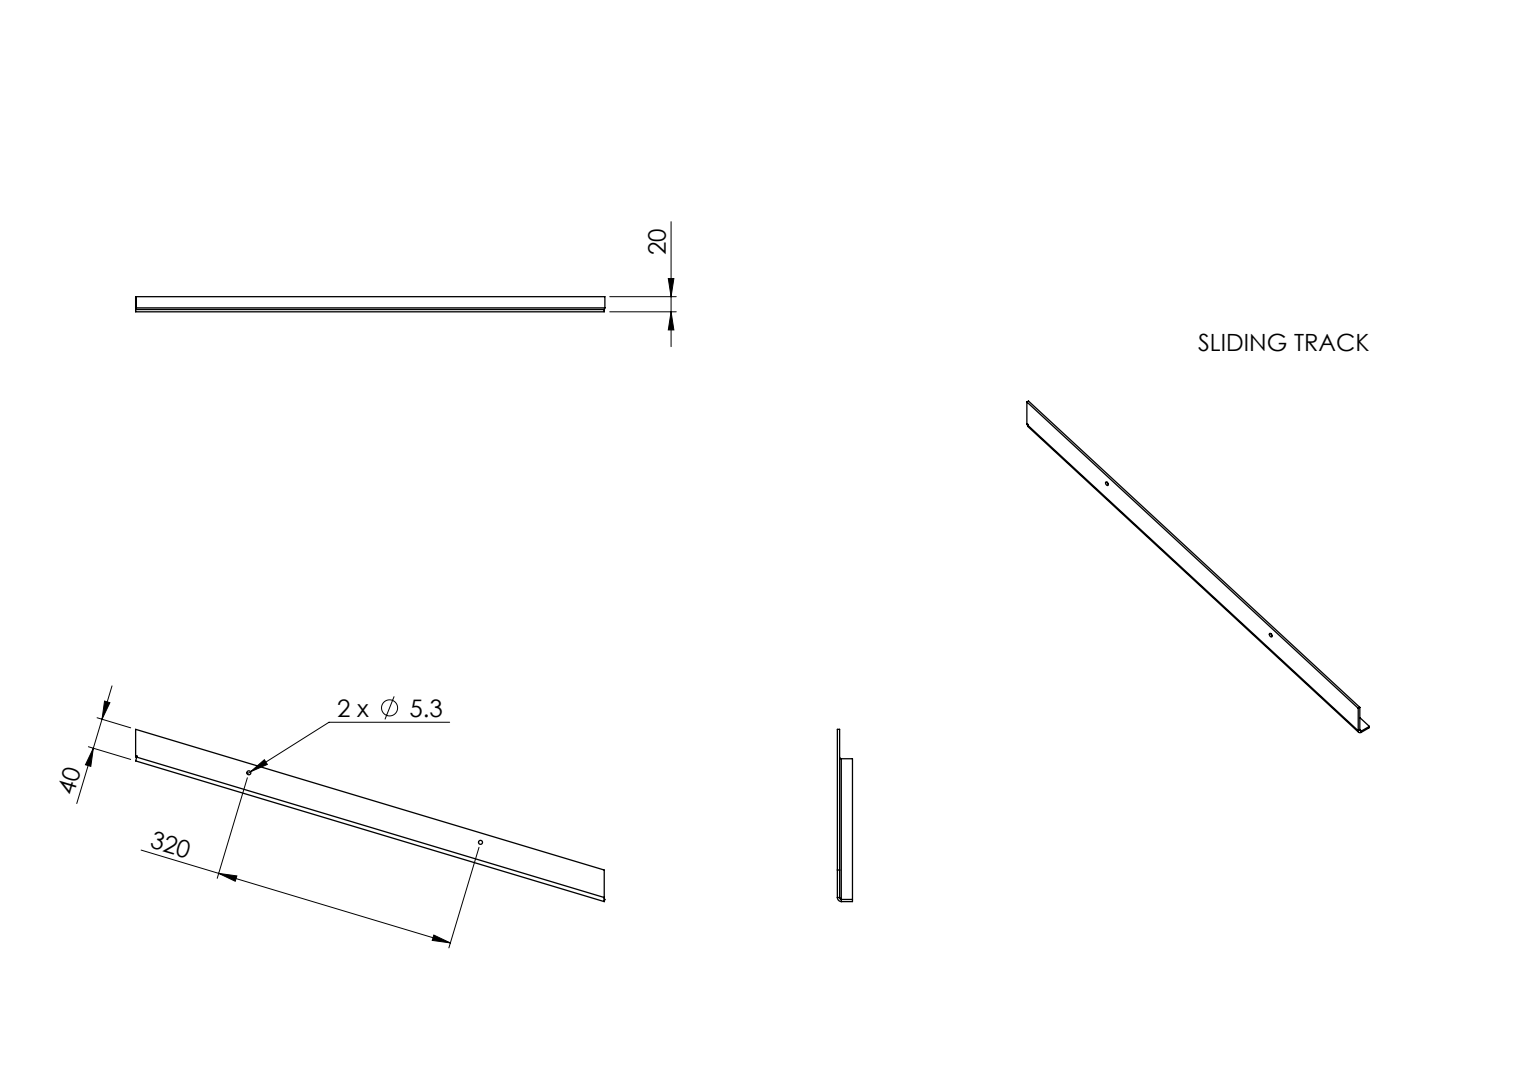
ISO-10303-21;
HEADER;
FILE_DESCRIPTION (('STEP AP214'),
    '1' );
FILE_NAME ('sliding track.step',
    '2026-10-27T17:01:19',
    ( '' ),
    ( '' ),
    'SwSTEP 2.0',
    'SolidWorks 2026',
    '' );
FILE_SCHEMA (( 'AUTOMOTIVE_DESIGN' ));
ENDSEC;

DATA;
#58=EDGE_CURVE ( 'NONE', #5396, #13410, #5058, .T. ) ;
#64=DIRECTION ( 'NONE',  ( 0.000000000000000000, 0.000000000000000000, 1.000000000000000000 ) ) ;
#77=EDGE_CURVE ( 'NONE', #2441, #3014, #1734, .T. ) ;
#96=SHAPE_REPRESENTATION_RELATIONSHIP ( 'NONE' , 'NONE' ,  #14430, #6538 ) ;
#102=ADVANCED_FACE ( 'NONE', ( #9327 ), #3935, .F. ) ;
#150=CARTESIAN_POINT ( 'NONE',  ( 142.4540310085880606, 355.9707293956415697, 187.0000000000000000 ) ) ;
#157=EDGE_CURVE ( 'NONE', #12209, #11318, #10435, .T. ) ;
#268=CARTESIAN_POINT ( 'NONE',  ( 610.0000000000001137, 185.6790804732684137, 184.8000000000000682 ) ) ;
#333=CARTESIAN_POINT ( 'NONE',  ( 609.8668404561643683, 185.6877074168924935, 185.4847245573741930 ) ) ;
#374=ORIENTED_EDGE ( 'NONE', *, *, #847, .F. ) ;
#378=DIRECTION ( 'NONE',  ( -1.000000000000000000, 0.000000000000000000, 0.000000000000000000 ) ) ;
#410=CARTESIAN_POINT ( 'NONE',  ( 609.6905198467529772, 186.4571330906553044, 187.4188186979287423 ) ) ;
#418=( GEOMETRIC_REPRESENTATION_CONTEXT ( 3 ) GLOBAL_UNCERTAINTY_ASSIGNED_CONTEXT ( ( #11082 ) ) GLOBAL_UNIT_ASSIGNED_CONTEXT ( ( #12770, #11436, #9372 ) ) REPRESENTATION_CONTEXT ( 'NONE', 'WORKASPACE' ) );
#467=DIRECTION ( 'NONE',  ( -0.9578262852211513190, 0.2873478855663453846, -8.575812866481462478E-17 ) ) ;
#511=DIRECTION ( 'NONE',  ( -1.000000000000000000, 0.000000000000000000, 0.000000000000000000 ) ) ;
#526=LINE ( 'NONE', #5051, #11486 ) ;
#558=CARTESIAN_POINT ( 'NONE',  ( 610.3687250539534261, 189.1718658564638247, 186.1427899493634470 ) ) ;
#572=ADVANCED_FACE ( 'NONE', ( #12850 ), #2893, .F. ) ;
#593=ORIENTED_EDGE ( 'NONE', *, *, #77, .F. ) ;
#627=CARTESIAN_POINT ( 'NONE',  ( -112.9080459801079144, 33.87241379403258890, 190.0000000000000000 ) ) ;
#629=CARTESIAN_POINT ( 'NONE',  ( 609.6990281814310038, 187.8427340524074225, 188.9822575857425022 ) ) ;
#644=VECTOR ( 'NONE', #4252, 1000.000000000000227 ) ;
#665=DIRECTION ( 'NONE',  ( -0.9578262852211518741, 0.2873478855663437748, 0.000000000000000000 ) ) ;
#688=AXIS2_PLACEMENT_3D ( 'NONE', #6223, #665, #7180 ) ;
#701=CARTESIAN_POINT ( 'NONE',  ( 610.0832774997078332, 190.4835367118463125, 186.9433982284626552 ) ) ;
#704=EDGE_CURVE ( 'NONE', #7308, #3640, #8632, .T. ) ;
#727=FACE_OUTER_BOUND ( 'NONE', #13601, .T. ) ;
#729=VECTOR ( 'NONE', #9292, 1000.000000000000000 ) ;
#743=CARTESIAN_POINT ( 'NONE',  ( 139.8040310085880833, 355.9707293956415697, 190.0000000000000000 ) ) ;
#847=EDGE_CURVE ( 'NONE', #13246, #3959, #4647, .T. ) ;
#913=CARTESIAN_POINT ( 'NONE',  ( 609.6836880993740806, 187.1145182921505921, 188.2379512264755874 ) ) ;
#933=AXIS2_PLACEMENT_3D ( 'NONE', #743, #5266, #12107 ) ;
#943=CARTESIAN_POINT ( 'NONE',  ( 610.0000000000000000, 227.4403065089105951, 187.0000000000000000 ) ) ;
#966=EDGE_CURVE ( 'NONE', #9351, #2398, #12904, .T. ) ;
#967=DIRECTION ( 'NONE',  ( -0.2873478855663452736, -0.9578262852211514300, 0.000000000000000000 ) ) ;
#979=ORIENTED_EDGE ( 'NONE', *, *, #13235, .T. ) ;
#981=CARTESIAN_POINT ( 'NONE',  ( 610.0000000000002274, 191.1080398579018720, 187.0000000000000284 ) ) ;
#983=VECTOR ( 'NONE', #4579, 1000.000000000000227 ) ;
#989=DIRECTION ( 'NONE',  ( 0.9578262852211513190, -0.2873478855663453846, -0.000000000000000000 ) ) ;
#993=CARTESIAN_POINT ( 'NONE',  ( 609.6939753585367043, 187.4861613156657540, 188.5968284039610978 ) ) ;
#1006=CARTESIAN_POINT ( 'NONE',  ( 610.1840840298345938, 189.9120001624725376, 186.6958543268122526 ) ) ;
#1011=EDGE_CURVE ( 'NONE', #2694, #5805, #12133, .T. ) ;
#1039=DIRECTION ( 'NONE',  ( 0.000000000000000000, -1.000000000000000000, 0.000000000000000000 ) ) ;
#1067=ORIENTED_EDGE ( 'NONE', *, *, #2953, .F. ) ;
#1077=( LENGTH_UNIT ( ) NAMED_UNIT ( * ) SI_UNIT ( .MILLI., .METRE. ) );
#1087=DIRECTION ( 'NONE',  ( -0.000000000000000000, 0.000000000000000000, 1.000000000000000000 ) ) ;
#1121=ORIENTED_EDGE ( 'NONE', *, *, #2407, .T. ) ;
#1142=AXIS2_PLACEMENT_3D ( 'NONE', #1745, #6320, #10822 ) ;
#1168=ORIENTED_EDGE ( 'NONE', *, *, #11531, .F. ) ;
#1171=PRODUCT_CONTEXT ( 'NONE', #13377, 'mechanical' ) ;
#1187=VECTOR ( 'NONE', #4576, 1000.000000000000000 ) ;
#1220=VECTOR ( 'NONE', #13865, 1000.000000000000114 ) ;
#1221=ORIENTED_EDGE ( 'NONE', *, *, #12699, .T. ) ;
#1323=CARTESIAN_POINT ( 'NONE',  ( 610.1812141201095301, 189.9029010627875493, 186.7093446292720387 ) ) ;
#1339=DIRECTION ( 'NONE',  ( -0.9578262852211514300, 0.2873478855663453846, -9.382948195091500646E-16 ) ) ;
#1366=DIRECTION ( 'NONE',  ( 1.000000000000000000, -0.000000000000000000, 0.000000000000000000 ) ) ;
#1377=DIRECTION ( 'NONE',  ( -0.2873478855663534892, -0.9578262852211489875, 0.000000000000000000 ) ) ;
#1445=( GEOMETRIC_REPRESENTATION_CONTEXT ( 3 ) GLOBAL_UNCERTAINTY_ASSIGNED_CONTEXT ( ( #5319 ) ) GLOBAL_UNIT_ASSIGNED_CONTEXT ( ( #1820, #9204, #5737 ) ) REPRESENTATION_CONTEXT ( 'NONE', 'WORKASPACE' ) );
#1463=ORIENTED_EDGE ( 'NONE', *, *, #9445, .F. ) ;
#1503=DIRECTION ( 'NONE',  ( 0.2873478855663453846, 0.9578262852211513190, 0.000000000000000000 ) ) ;
#1514=CYLINDRICAL_SURFACE ( 'NONE', #14409, 2.649999999999985700 ) ;
#1534=CARTESIAN_POINT ( 'NONE',  ( 609.7043258424479291, 187.8603929224640581, 188.9582675804705332 ) ) ;
#1560=ADVANCED_FACE ( 'NONE', ( #5549 ), #14553, .F. ) ;
#1564=CARTESIAN_POINT ( 'NONE',  ( -8.505790995055050985, 376.6597771564184995, 184.8000000000000398 ) ) ;
#1575=LINE ( 'NONE', #4915, #1681 ) ;
#1585=DIRECTION ( 'NONE',  ( 0.2873478855663471054, 0.9578262852211508749, 1.632680918566126195E-14 ) ) ;
#1600=ORIENTED_EDGE ( 'NONE', *, *, #10084, .F. ) ;
#1601=CARTESIAN_POINT ( 'NONE',  ( 609.7412162373094588, 188.4357741873886880, 189.3699028110927429 ) ) ;
#1611=MECHANICAL_DESIGN_GEOMETRIC_PRESENTATION_REPRESENTATION('',(#13870),#418);
#1612=DIRECTION ( 'NONE',  ( -0.000000000000000000, -0.000000000000000000, -1.000000000000000000 ) ) ;
#1641=EDGE_LOOP ( 'NONE', ( #4198, #14567, #10049, #8130 ) ) ;
#1666=DIRECTION ( 'NONE',  ( 0.2873478855663452736, 0.9578262852211513190, -3.491481338843133355E-15 ) ) ;
#1681=VECTOR ( 'NONE', #467, 1000.000000000000114 ) ;
#1686=CARTESIAN_POINT ( 'NONE',  ( 609.8754609228352592, 185.7164421964179439, 185.4807968138250374 ) ) ;
#1733=DIRECTION ( 'NONE',  ( 0.000000000000000000, 0.000000000000000000, 1.000000000000000000 ) ) ;
#1734=CIRCLE ( 'NONE', #12322, 2.649999999999985700 ) ;
#1745=CARTESIAN_POINT ( 'NONE',  ( 139.8040310085880833, 355.9707293956415697, 187.0000000000000000 ) ) ;
#1791=CARTESIAN_POINT ( 'NONE',  ( -10.00000000000000000, 371.6790804732683569, 187.0000000000000000 ) ) ;
#1808=CARTESIAN_POINT ( 'NONE',  ( 443.6584422793565636, 264.0194060144110608, 187.0000000000000000 ) ) ;
#1820=( LENGTH_UNIT ( ) NAMED_UNIT ( * ) SI_UNIT ( .MILLI., .METRE. ) );
#1826=EDGE_LOOP ( 'NONE', ( #9063, #13172, #6884, #1878 ) ) ;
#1830=FACE_BOUND ( 'NONE', #8586, .T. ) ;
#1878=ORIENTED_EDGE ( 'NONE', *, *, #11509, .T. ) ;
#1888=CARTESIAN_POINT ( 'NONE',  ( 609.7983275391768530, 185.9141716657875349, 186.1519484124941641 ) ) ;
#1898=DIRECTION ( 'NONE',  ( 0.9578262852211513190, -0.2873478855663453846, -0.000000000000000000 ) ) ;
#1909=ORIENTED_EDGE ( 'NONE', *, *, #2407, .F. ) ;
#1928=ORIENTED_EDGE ( 'NONE', *, *, #5544, .T. ) ;
#2001=EDGE_LOOP ( 'NONE', ( #13223, #10824, #12086, #8874 ) ) ;
#2009=EDGE_LOOP ( 'NONE', ( #7216, #9637, #10310, #9166 ) ) ;
#2023=CARTESIAN_POINT ( 'NONE',  ( 609.8615525982525014, 189.7413297629623514, 189.8335177487570888 ) ) ;
#2076=DIRECTION ( 'NONE',  ( -8.745957808406929547E-15, -2.915319269468972624E-14, 1.000000000000000000 ) ) ;
#2140=CARTESIAN_POINT ( 'NONE',  ( -111.4713065522750952, 33.44139196568231398, 190.0000000000000000 ) ) ;
#2156=ORIENTED_EDGE ( 'NONE', *, *, #13907, .F. ) ;
#2166=ORIENTED_EDGE ( 'NONE', *, *, #9445, .T. ) ;
#2213=CARTESIAN_POINT ( 'NONE',  ( 610.0000000000000000, 227.4403065089105951, 187.0000000000000000 ) ) ;
#2233=ORIENTED_EDGE ( 'NONE', *, *, #8909, .T. ) ;
#2261=CARTESIAN_POINT ( 'NONE',  ( -9.137956343300997375, 374.5525593289318635, 169.9999999999999716 ) ) ;
#2262=ADVANCED_FACE ( 'NONE', ( #10592 ), #14138, .T. ) ;
#2263=CARTESIAN_POINT ( 'NONE',  ( 137.1540310085880776, 355.9707293956415697, 187.0000000000000000 ) ) ;
#2327=SURFACE_STYLE_FILL_AREA ( #10166 ) ;
#2335=CARTESIAN_POINT ( 'NONE',  ( -9.511508594537124495, 378.5275384125996538, 187.0000000000000284 ) ) ;
#2366=DIRECTION ( 'NONE',  ( -0.000000000000000000, -0.000000000000000000, -1.000000000000000000 ) ) ;
#2383=DIRECTION ( 'NONE',  ( -9.028085479645851510E-15, -3.009361826548617065E-14, 1.000000000000000000 ) ) ;
#2398=VERTEX_POINT ( 'NONE', #5265 ) ;
#2407=EDGE_CURVE ( 'NONE', #3959, #8752, #526, .T. ) ;
#2415=FILL_AREA_STYLE_COLOUR ( '', #3334 ) ;
#2421=EDGE_LOOP ( 'NONE', ( #9229, #7654, #3804, #9012 ) ) ;
#2422=FACE_OUTER_BOUND ( 'NONE', #12765, .T. ) ;
#2429=EDGE_CURVE ( 'NONE', #7308, #13410, #10782, .T. ) ;
#2436=CARTESIAN_POINT ( 'NONE',  ( 610.4468987511024807, 188.9818594558784355, 185.9044171606945497 ) ) ;
#2441=VERTEX_POINT ( 'NONE', #14329 ) ;
#2475=FACE_OUTER_BOUND ( 'NONE', #3623, .T. ) ;
#2480=ORIENTED_EDGE ( 'NONE', *, *, #9254, .F. ) ;
#2501=EDGE_LOOP ( 'NONE', ( #8907, #593, #7904, #13270 ) ) ;
#2537=ORIENTED_EDGE ( 'NONE', *, *, #58, .T. ) ;
#2552=VECTOR ( 'NONE', #5814, 1000.000000000000227 ) ;
#2556=B_SPLINE_CURVE_WITH_KNOTS ( 'NONE', 3,
 ( #4333, #6613, #13325, #2023, #7717, #8887, #11114, #8606, #7494, #9939, #993, #913, #5356, #3154, #7656, #2996, #1888, #7579, #11991, #14290 ),
 .UNSPECIFIED., .F., .F.,
 ( 4, 2, 2, 2, 2, 2, 2, 2, 2, 4 ),
 ( 5.551115123125782702E-17, 0.001037574205614438111, 0.002075148411228820711, 0.003112722616843203310, 0.003631509719650373360, 0.004150296822457543409, 0.005187871028071766415, 0.006225445233685987685, 0.007263019439300210690, 0.008300593644914432828 ),
 .UNSPECIFIED. ) ;
#2565=VERTEX_POINT ( 'NONE', #10997 ) ;
#2571=ORIENTED_EDGE ( 'NONE', *, *, #8909, .F. ) ;
#2617=MANIFOLD_SOLID_BREP ( 'M5 Clearance Hole1', #11159 ) ;
#2684=FACE_OUTER_BOUND ( 'NONE', #1826, .T. ) ;
#2694=VERTEX_POINT ( 'NONE', #8561 ) ;
#2703=CARTESIAN_POINT ( 'NONE',  ( -10.00000000000000000, 371.6790804732683569, 187.0000000000000000 ) ) ;
#2708=EDGE_LOOP ( 'NONE', ( #12529, #3000, #13955, #4120 ) ) ;
#2731=DIRECTION ( 'NONE',  ( -0.000000000000000000, -0.000000000000000000, -1.000000000000000000 ) ) ;
#2783=VECTOR ( 'NONE', #989, 1000.000000000000114 ) ;
#2785=CARTESIAN_POINT ( 'NONE',  ( 609.9277849535120595, 190.4148309465319358, 190.0300000000000296 ) ) ;
#2796=AXIS2_PLACEMENT_3D ( 'NONE', #9839, #4020, #3053 ) ;
#2814=FACE_OUTER_BOUND ( 'NONE', #11072, .T. ) ;
#2817=CARTESIAN_POINT ( 'NONE',  ( -9.511508594537124495, 378.5275384125996538, 187.0000000000000284 ) ) ;
#2870=VERTEX_POINT ( 'NONE', #6425 ) ;
#2890=PRODUCT_DEFINITION_SHAPE ( 'NONE', 'NONE',  #13442 ) ;
#2893=CYLINDRICAL_SURFACE ( 'NONE', #9310, 2.649999999999985700 ) ;
#2953=EDGE_CURVE ( 'NONE', #2565, #13081, #9395, .T. ) ;
#2959=ADVANCED_FACE ( 'NONE', ( #2422 ), #10174, .T. ) ;
#2996=CARTESIAN_POINT ( 'NONE',  ( 609.7645211877446627, 186.0291131959509698, 186.4810828243464016 ) ) ;
#3000=ORIENTED_EDGE ( 'NONE', *, *, #5185, .T. ) ;
#3006=DIRECTION ( 'NONE',  ( -0.2873478855663470499, -0.9578262852211508749, 0.000000000000000000 ) ) ;
#3014=VERTEX_POINT ( 'NONE', #9288 ) ;
#3029=AXIS2_PLACEMENT_3D ( 'NONE', #5882, #13719, #12667 ) ;
#3053=DIRECTION ( 'NONE',  ( 0.9578262852211513190, -0.2873478855663453846, 0.000000000000000000 ) ) ;
#3070=LINE ( 'NONE', #13256, #8958 ) ;
#3081=CIRCLE ( 'NONE', #13212, 2.649999999999985700 ) ;
#3087=VECTOR ( 'NONE', #4355, 1000.000000000000000 ) ;
#3106=CIRCLE ( 'NONE', #7104, 2.649999999999985700 ) ;
#3107=PRODUCT_DEFINITION_CONTEXT ( 'detailed design', #7544, 'design' ) ;
#3139=CARTESIAN_POINT ( 'NONE',  ( -8.505790995054914205, 376.6597771564183859, 187.0000000000000284 ) ) ;
#3154=CARTESIAN_POINT ( 'NONE',  ( 609.6994022290995190, 186.4862707338506311, 187.4054488658613593 ) ) ;
#3222=EDGE_CURVE ( 'NONE', #11200, #5805, #13535, .T. ) ;
#3284=LINE ( 'NONE', #150, #13745 ) ;
#3312=VECTOR ( 'NONE', #4594, 1000.000000000000114 ) ;
#3317=LINE ( 'NONE', #2261, #3087 ) ;
#3334=COLOUR_RGB ( '',0.8941176470588234615, 0.8941176470588234615, 0.8941176470588234615 ) ;
#3413=EDGE_LOOP ( 'NONE', ( #11370, #10060, #9371, #14454 ) ) ;
#3414=EDGE_CURVE ( 'NONE', #3596, #7551, #11604, .T. ) ;
#3519=ORIENTED_EDGE ( 'NONE', *, *, #4856, .F. ) ;
#3545=CARTESIAN_POINT ( 'NONE',  ( 610.8620436566991430, 188.5525593289319488, 184.8000000000000398 ) ) ;
#3549=LINE ( 'NONE', #4740, #4279 ) ;
#3596=VERTEX_POINT ( 'NONE', #2213 ) ;
#3623=EDGE_LOOP ( 'NONE', ( #2233, #10282, #12724, #12370 ) ) ;
#3640=VERTEX_POINT ( 'NONE', #7690 ) ;
#3666=CARTESIAN_POINT ( 'NONE',  ( 610.0000000000001137, 191.1080398579018720, 190.0000000000000000 ) ) ;
#3672=ADVANCED_FACE ( 'NONE', ( #5480 ), #12250, .F. ) ;
#3709=PLANE ( 'NONE',  #11986 ) ;
#3734=CARTESIAN_POINT ( 'NONE',  ( 446.3084422793565409, 264.0194060144110608, 187.0000000000000000 ) ) ;
#3744=VECTOR ( 'NONE', #1039, 1000.000000000000000 ) ;
#3758=CARTESIAN_POINT ( 'NONE',  ( 610.0000000000001137, 191.1080398579019288, 190.0000000000000284 ) ) ;
#3788=DIRECTION ( 'NONE',  ( -0.000000000000000000, -0.000000000000000000, 1.000000000000000000 ) ) ;
#3804=ORIENTED_EDGE ( 'NONE', *, *, #3414, .T. ) ;
#3823=DIRECTION ( 'NONE',  ( 0.9578262852211508749, -0.2873478855663470499, 0.000000000000000000 ) ) ;
#3845=PRODUCT_DEFINITION_FORMATION_WITH_SPECIFIED_SOURCE ( 'ANY', '', #8160, .NOT_KNOWN. ) ;
#3848=EDGE_CURVE ( 'NONE', #9351, #13246, #9532, .T. ) ;
#3870=DIRECTION ( 'NONE',  ( -0.000000000000000000, -0.000000000000000000, -1.000000000000000000 ) ) ;
#3877=DIRECTION ( 'NONE',  ( -0.000000000000000000, -0.000000000000000000, -1.000000000000000000 ) ) ;
#3912=ORIENTED_EDGE ( 'NONE', *, *, #13781, .T. ) ;
#3917=PLANE ( 'NONE',  #11757 ) ;
#3919=ADVANCED_FACE ( 'NONE', ( #1830, #5315, #727 ), #3917, .F. ) ;
#3935=CYLINDRICAL_SURFACE ( 'NONE', #4310, 2.199999999999984635 ) ;
#3959=VERTEX_POINT ( 'NONE', #12158 ) ;
#3975=CARTESIAN_POINT ( 'NONE',  ( 610.4437618601435815, 188.9679398019578116, 185.9079617568160074 ) ) ;
#3984=CIRCLE ( 'NONE', #4696, 2.649999999999985700 ) ;
#4006=VECTOR ( 'NONE', #4070, 1000.000000000000000 ) ;
#4020=DIRECTION ( 'NONE',  ( -0.2873478855663454401, -0.9578262852211514300, 0.000000000000000000 ) ) ;
#4070=DIRECTION ( 'NONE',  ( -2.449021377849607626E-15, -3.265361837132810036E-15, -1.000000000000000000 ) ) ;
#4095=VECTOR ( 'NONE', #12798, 1000.000000000000114 ) ;
#4120=ORIENTED_EDGE ( 'NONE', *, *, #3848, .F. ) ;
#4121=ORIENTED_EDGE ( 'NONE', *, *, #12555, .T. ) ;
#4167=ORIENTED_EDGE ( 'NONE', *, *, #13136, .T. ) ;
#4198=ORIENTED_EDGE ( 'NONE', *, *, #157, .F. ) ;
#4202=CARTESIAN_POINT ( 'NONE',  ( -10.00000000000045297, 371.6790804732678453, -1.178702027242996938E-12 ) ) ;
#4247=AXIS2_PLACEMENT_3D ( 'NONE', #2703, #1366, #6019 ) ;
#4252=DIRECTION ( 'NONE',  ( -0.2873478855663453291, -0.9578262852211513190, 3.835990623682899812E-15 ) ) ;
#4269=CARTESIAN_POINT ( 'NONE',  ( 610.7462142612635034, 188.6189422762846561, 185.0840554379255707 ) ) ;
#4279=VECTOR ( 'NONE', #1612, 1000.000000000000000 ) ;
#4310=AXIS2_PLACEMENT_3D ( 'NONE', #1564, #4983, #13823 ) ;
#4332=ORIENTED_EDGE ( 'NONE', *, *, #13781, .F. ) ;
#4333=CARTESIAN_POINT ( 'NONE',  ( 610.0000000000001137, 191.1080398579018720, 190.0000000000000000 ) ) ;
#4347=CARTESIAN_POINT ( 'NONE',  ( 0.000000000000000000, 0.000000000000000000, 0.000000000000000000 ) ) ;
#4355=DIRECTION ( 'NONE',  ( -2.449021377849607626E-15, -3.265361837132810036E-15, -1.000000000000000000 ) ) ;
#4387=ORIENTED_EDGE ( 'NONE', *, *, #10706, .F. ) ;
#4419=AXIS2_PLACEMENT_3D ( 'NONE', #13926, #3823, #14067 ) ;
#4444=CARTESIAN_POINT ( 'NONE',  ( 446.3084422793565409, 264.0194060144110608, 187.0000000000000000 ) ) ;
#4455=CARTESIAN_POINT ( 'NONE',  ( 610.0000000000000000, 227.4403065089105951, 190.0000000000000000 ) ) ;
#4508=CARTESIAN_POINT ( 'NONE',  ( 101.4713065522757063, 338.2376885075856876, 169.9999999999999716 ) ) ;
#4524=B_SPLINE_SURFACE_WITH_KNOTS ( 'NONE', 1, 3, ( 
 ( #11703, #2785, #10471, #1601, #629, #7149, #7286, #14019, #333, #9361 ),
 ( #3758, #8244, #7217, #12757, #1534, #9437, #410, #8390, #1686, #13946 ),
 ( #5153, #6115, #6193, #10691, #5087, #9583, #3975, #7368, #9659, #11125 ),
 ( #14299, #13057, #7507, #1006, #14373, #10913, #5237, #8773, #4269, #7590 ) ),
 .UNSPECIFIED., .F., .F., .F.,
 ( 2, 1, 1, 2 ),
 ( 4, 2, 2, 2, 4 ),
 ( -0.01000000000000000021, 0.000000000000000000, 1.000000000000000000, 1.010099999999999998 ),
 ( 0.000000000000000000, 0.2500000000000000000, 0.5000000000000000000, 0.7500000000000000000, 1.000000000000000000 ),
 .UNSPECIFIED. ) ;
#4568=( NAMED_UNIT ( * ) PLANE_ANGLE_UNIT ( ) SI_UNIT ( $, .RADIAN. ) );
#4576=DIRECTION ( 'NONE',  ( 2.022127743178574844E-16, 3.939404418192334771E-15, 1.000000000000000000 ) ) ;
#4579=DIRECTION ( 'NONE',  ( -0.2873478855663453291, -0.9578262852211513190, 3.835990623682899812E-15 ) ) ;
#4594=DIRECTION ( 'NONE',  ( 0.2873478855663437748, 0.9578262852211518741, 0.000000000000000000 ) ) ;
#4605=CARTESIAN_POINT ( 'NONE',  ( 446.3084422793565409, 264.0194060144110608, 187.0000000000000000 ) ) ;
#4634=( NAMED_UNIT ( * ) SI_UNIT ( $, .STERADIAN. ) SOLID_ANGLE_UNIT ( ) );
#4647=LINE ( 'NONE', #4508, #2552 ) ;
#4696=AXIS2_PLACEMENT_3D ( 'NONE', #4605, #13667, #11381 ) ;
#4729=EDGE_CURVE ( 'NONE', #12823, #5137, #11905, .T. ) ;
#4740=CARTESIAN_POINT ( 'NONE',  ( 448.9584422793565750, 264.0194060144110608, 187.0000000000000000 ) ) ;
#4759=PLANE ( 'NONE',  #6385 ) ;
#4774=CARTESIAN_POINT ( 'NONE',  ( -8.505790995055050985, 376.6597771564184995, 184.8000000000000398 ) ) ;
#4780=ORIENTED_EDGE ( 'NONE', *, *, #2429, .T. ) ;
#4836=PLANE ( 'NONE',  #9429 ) ;
#4845=ORIENTED_EDGE ( 'NONE', *, *, #13136, .F. ) ;
#4856=EDGE_CURVE ( 'NONE', #7551, #5805, #5500, .T. ) ;
#4890=FACE_OUTER_BOUND ( 'NONE', #11371, .T. ) ;
#4915=CARTESIAN_POINT ( 'NONE',  ( 610.8620436566991430, 188.5525593289318920, 184.8000000000000682 ) ) ;
#4925=AXIS2_PLACEMENT_3D ( 'NONE', #2335, #1377, #10392 ) ;
#4938=EDGE_LOOP ( 'NONE', ( #4780, #1928, #2571, #3912 ) ) ;
#4954=ORIENTED_EDGE ( 'NONE', *, *, #9632, .F. ) ;
#4968=CARTESIAN_POINT ( 'NONE',  ( -9.999999999999957367, 376.8992337277236970, 190.0000000000000000 ) ) ;
#4983=DIRECTION ( 'NONE',  ( -0.9578262852211514300, 0.2873478855663454401, 0.000000000000000000 ) ) ;
#4988=DIRECTION ( 'NONE',  ( -0.2873478855663446629, -0.9578262852211516520, 5.337610695313252962E-15 ) ) ;
#4996=CARTESIAN_POINT ( 'NONE',  ( 610.0000000000002274, 185.6790804732676747, -8.443403382996446544E-13 ) ) ;
#5007=PLANE ( 'NONE',  #4247 ) ;
#5046=CARTESIAN_POINT ( 'NONE',  ( -10.00000000000000000, 413.4403065089105667, 187.0000000000000000 ) ) ;
#5051=CARTESIAN_POINT ( 'NONE',  ( 610.0000000000001137, 185.6790804732683853, 169.9999999999999716 ) ) ;
#5058=LINE ( 'NONE', #9484, #4095 ) ;
#5087=CARTESIAN_POINT ( 'NONE',  ( 610.2340919441475080, 189.6262799281293212, 186.5592670532760167 ) ) ;
#5118=FACE_OUTER_BOUND ( 'NONE', #2421, .T. ) ;
#5127=ORIENTED_EDGE ( 'NONE', *, *, #9254, .T. ) ;
#5137=VERTEX_POINT ( 'NONE', #6267 ) ;
#5146=CARTESIAN_POINT ( 'NONE',  ( 610.4899793196105975, 188.8968529749589038, 185.7755421771552165 ) ) ;
#5153=CARTESIAN_POINT ( 'NONE',  ( 610.0000000000001137, 191.1080398579019572, 187.0000000000000284 ) ) ;
#5185=EDGE_CURVE ( 'NONE', #12209, #12104, #3317, .T. ) ;
#5215=EDGE_CURVE ( 'NONE', #8752, #2870, #7822, .T. ) ;
#5226=( GEOMETRIC_REPRESENTATION_CONTEXT ( 3 ) GLOBAL_UNCERTAINTY_ASSIGNED_CONTEXT ( ( #8406 ) ) GLOBAL_UNIT_ASSIGNED_CONTEXT ( ( #1077, #4568, #4634 ) ) REPRESENTATION_CONTEXT ( 'NONE', 'WORKASPACE' ) );
#5228=DIRECTION ( 'NONE',  ( 0.9578262852211513190, -0.2873478855663453291, -0.000000000000000000 ) ) ;
#5237=CARTESIAN_POINT ( 'NONE',  ( 610.4513696044788276, 188.9932989497419555, 185.8927021017107677 ) ) ;
#5265=CARTESIAN_POINT ( 'NONE',  ( 610.0000000000001137, 185.6790804732684705, 184.8000000000000398 ) ) ;
#5266=DIRECTION ( 'NONE',  ( -0.000000000000000000, -0.000000000000000000, -1.000000000000000000 ) ) ;
#5296=CARTESIAN_POINT ( 'NONE',  ( -10.00000000000004263, 371.6790804732683569, 169.9999999999999716 ) ) ;
#5309=ORIENTED_EDGE ( 'NONE', *, *, #5528, .T. ) ;
#5315=FACE_BOUND ( 'NONE', #11191, .T. ) ;
#5319=UNCERTAINTY_MEASURE_WITH_UNIT (LENGTH_MEASURE( 1.000000000000000082E-05 ), #1820, 'distance_accuracy_value', 'NONE');
#5356=CARTESIAN_POINT ( 'NONE',  ( 609.6834941627989792, 186.8890602495695248, 187.9755619318007405 ) ) ;
#5370=DIRECTION ( 'NONE',  ( -0.000000000000000000, -0.000000000000000000, -1.000000000000000000 ) ) ;
#5396=VERTEX_POINT ( 'NONE', #6987 ) ;
#5403=VECTOR ( 'NONE', #5228, 1000.000000000000114 ) ;
#5412=DIRECTION ( 'NONE',  ( 0.000000000000000000, 1.000000000000000000, 0.000000000000000000 ) ) ;
#5438=EDGE_LOOP ( 'NONE', ( #11345, #1067 ) ) ;
#5480=FACE_OUTER_BOUND ( 'NONE', #3413, .T. ) ;
#5500=LINE ( 'NONE', #4455, #10384 ) ;
#5528=EDGE_CURVE ( 'NONE', #3014, #2441, #13709, .T. ) ;
#5537=SHAPE_DEFINITION_REPRESENTATION ( #2890, #14430 ) ;
#5544=EDGE_CURVE ( 'NONE', #13410, #12823, #10751, .T. ) ;
#5549=FACE_OUTER_BOUND ( 'NONE', #2501, .T. ) ;
#5550=CARTESIAN_POINT ( 'NONE',  ( -8.074769166705396017, 378.0965165842501392, 187.0000000000000284 ) ) ;
#5556=DIRECTION ( 'NONE',  ( -0.000000000000000000, -0.000000000000000000, -1.000000000000000000 ) ) ;
#5609=ORIENTED_EDGE ( 'NONE', *, *, #9595, .T. ) ;
#5697=VECTOR ( 'NONE', #5947, 1000.000000000000000 ) ;
#5737=( NAMED_UNIT ( * ) SI_UNIT ( $, .STERADIAN. ) SOLID_ANGLE_UNIT ( ) );
#5776=DIRECTION ( 'NONE',  ( -0.2873478855663446629, -0.9578262852211516520, 0.000000000000000000 ) ) ;
#5779=EDGE_LOOP ( 'NONE', ( #7767, #4332, #10904, #979, #6233, #4387, #9042 ) ) ;
#5781=CARTESIAN_POINT ( 'NONE',  ( 610.0000000000001137, 191.1080398579018720, 187.0000000000000000 ) ) ;
#5805=VERTEX_POINT ( 'NONE', #3666 ) ;
#5814=DIRECTION ( 'NONE',  ( 0.9578262852211513190, -0.2873478855663454401, 1.972152263052529951E-31 ) ) ;
#5818=CARTESIAN_POINT ( 'NONE',  ( 610.5828669213532294, 188.7537838752662935, 185.5093481647506906 ) ) ;
#5829=CARTESIAN_POINT ( 'NONE',  ( 610.8620436566991430, 188.5525593289318351, 169.9999999999999716 ) ) ;
#5840=ORIENTED_EDGE ( 'NONE', *, *, #7446, .T. ) ;
#5854=DIRECTION ( 'NONE',  ( -0.000000000000000000, -0.000000000000000000, -1.000000000000000000 ) ) ;
#5882=CARTESIAN_POINT ( 'NONE',  ( 446.3084422793565409, 264.0194060144110608, 187.0000000000000000 ) ) ;
#5910=LINE ( 'NONE', #5829, #7803 ) ;
#5947=DIRECTION ( 'NONE',  ( 2.022127743178574844E-16, 3.939404418192334771E-15, 1.000000000000000000 ) ) ;
#5964=EDGE_LOOP ( 'NONE', ( #12286, #9782, #13998, #1221 ) ) ;
#5986=CARTESIAN_POINT ( 'NONE',  ( 139.8040310085880833, 355.9707293956415697, 187.0000000000000000 ) ) ;
#5997=CARTESIAN_POINT ( 'NONE',  ( 610.0000000000000000, 227.4403065089105951, 187.0000000000000000 ) ) ;
#6002=FACE_OUTER_BOUND ( 'NONE', #1641, .T. ) ;
#6005=DIRECTION ( 'NONE',  ( -0.9578262852211514300, 0.2873478855663454401, 0.000000000000000000 ) ) ;
#6019=DIRECTION ( 'NONE',  ( 0.000000000000000000, 0.000000000000000000, -1.000000000000000000 ) ) ;
#6059=DIRECTION ( 'NONE',  ( -0.2873478855663453291, -0.9578262852211513190, 0.000000000000000000 ) ) ;
#6065=CARTESIAN_POINT ( 'NONE',  ( -10.00000000000002487, 371.6790804732684705, 184.8000000000000114 ) ) ;
#6066=B_SPLINE_CURVE_WITH_KNOTS ( 'NONE', 3,
 ( #13049, #11497, #701, #6934, #1323, #12614, #9143, #11853, #558, #2436, #5146, #5818, #14152, #7277, #13649, #3545 ),
 .UNSPECIFIED., .F., .F.,
 ( 4, 2, 2, 2, 2, 2, 2, 4 ),
 ( 8.777083671441753062E-17, 0.0009429092714760194203, 0.001414363907214010374, 0.001885818542952001327, 0.002357273178689992064, 0.002828727814427983017, 0.003300182450165973971, 0.003771637085903964924 ),
 .UNSPECIFIED. ) ;
#6075=CARTESIAN_POINT ( 'NONE',  ( -8.505790995054926640, 376.6597771564183859, 187.0000000000000000 ) ) ;
#6115=CARTESIAN_POINT ( 'NONE',  ( 610.0417734222098716, 190.7948035559919333, 187.0000000000000284 ) ) ;
#6167=ORIENTED_EDGE ( 'NONE', *, *, #5544, .F. ) ;
#6193=CARTESIAN_POINT ( 'NONE',  ( 610.0835668916889745, 190.4817695994259736, 186.9427398886703315 ) ) ;
#6223=CARTESIAN_POINT ( 'NONE',  ( -8.074769166705396017, 378.0965165842501392, 187.0000000000000284 ) ) ;
#6233=ORIENTED_EDGE ( 'NONE', *, *, #12631, .T. ) ;
#6267=CARTESIAN_POINT ( 'NONE',  ( -10.00000000000000000, 413.4403065089105667, 190.0000000000000000 ) ) ;
#6320=DIRECTION ( 'NONE',  ( -0.000000000000000000, -0.000000000000000000, -1.000000000000000000 ) ) ;
#6325=CARTESIAN_POINT ( 'NONE',  ( 446.3084422793565409, 264.0194060144110608, 190.0000000000000000 ) ) ;
#6357=VERTEX_POINT ( 'NONE', #7353 ) ;
#6376=CARTESIAN_POINT ( 'NONE',  ( 142.4540310085880606, 355.9707293956415697, 190.0000000000000000 ) ) ;
#6385=AXIS2_PLACEMENT_3D ( 'NONE', #11519, #1339, #6059 ) ;
#6417=DIRECTION ( 'NONE',  ( 1.000000000000000000, 0.000000000000000000, 0.000000000000000000 ) ) ;
#6425=CARTESIAN_POINT ( 'NONE',  ( 610.8620436566991430, 188.5525593289319488, 184.8000000000000398 ) ) ;
#6437=AXIS2_PLACEMENT_3D ( 'NONE', #12152, #11045, #14240 ) ;
#6463=EDGE_CURVE ( 'NONE', #12209, #9351, #13107, .T. ) ;
#6488=LINE ( 'NONE', #10977, #12550 ) ;
#6534=CARTESIAN_POINT ( 'NONE',  ( -9.137956343300945861, 374.5525593289318635, 184.8000000000000114 ) ) ;
#6538=ADVANCED_BREP_SHAPE_REPRESENTATION ( '', ( #2617, #9440 ), #1445 ) ;
#6549=CARTESIAN_POINT ( 'NONE',  ( -9.511508594537115613, 378.5275384125997107, 190.0000000000000000 ) ) ;
#6580=CARTESIAN_POINT ( 'NONE',  ( 101.4713065522755215, 338.2376885075850623, -1.342499394901007523E-12 ) ) ;
#6592=AXIS2_PLACEMENT_3D ( 'NONE', #6580, #6791, #11154 ) ;
#6613=CARTESIAN_POINT ( 'NONE',  ( 609.9641659369621038, 190.7604956903689413, 190.0000000000000568 ) ) ;
#6639=VECTOR ( 'NONE', #3006, 1000.000000000000114 ) ;
#6699=FACE_BOUND ( 'NONE', #12909, .T. ) ;
#6703=ADVANCED_FACE ( 'NONE', ( #11460 ), #13764, .T. ) ;
#6734=ORIENTED_EDGE ( 'NONE', *, *, #9595, .F. ) ;
#6736=CARTESIAN_POINT ( 'NONE',  ( 139.8040310085880833, 355.9707293956415697, 187.0000000000000000 ) ) ;
#6791=DIRECTION ( 'NONE',  ( 0.2873478855663454401, 0.9578262852211514300, -3.831370512995697396E-15 ) ) ;
#6826=CARTESIAN_POINT ( 'NONE',  ( 610.8620436566991430, 188.5525593289318351, 169.9999999999999716 ) ) ;
#6843=CARTESIAN_POINT ( 'NONE',  ( -9.511508594537115613, 378.5275384125997107, 187.0000000000000000 ) ) ;
#6858=VERTEX_POINT ( 'NONE', #8655 ) ;
#6874=DIRECTION ( 'NONE',  ( -1.000000000000000000, 0.000000000000000000, 0.000000000000000000 ) ) ;
#6879=CARTESIAN_POINT ( 'NONE',  ( 610.0000000000000000, 227.4403065089105951, 187.0000000000000000 ) ) ;
#6884=ORIENTED_EDGE ( 'NONE', *, *, #12555, .F. ) ;
#6934=CARTESIAN_POINT ( 'NONE',  ( 610.1557962250110450, 190.0426856094898085, 186.7771368031600048 ) ) ;
#6987=CARTESIAN_POINT ( 'NONE',  ( -8.074769166705394241, 378.0965165842501392, 190.0000000000000000 ) ) ;
#6988=ORIENTED_EDGE ( 'NONE', *, *, #704, .T. ) ;
#7076=AXIS2_PLACEMENT_3D ( 'NONE', #12033, #11951, #7624 ) ;
#7104=AXIS2_PLACEMENT_3D ( 'NONE', #6736, #5556, #10211 ) ;
#7128=DIRECTION ( 'NONE',  ( 0.000000000000000000, 1.000000000000000000, 0.000000000000000000 ) ) ;
#7149=CARTESIAN_POINT ( 'NONE',  ( 609.6698590453944462, 186.8406770348469195, 188.0140793454688151 ) ) ;
#7180=DIRECTION ( 'NONE',  ( -0.2873478855663437748, -0.9578262852211518741, 0.000000000000000000 ) ) ;
#7184=CARTESIAN_POINT ( 'NONE',  ( -8.505790995054899994, 376.6597771564184427, 184.8000000000000398 ) ) ;
#7216=ORIENTED_EDGE ( 'NONE', *, *, #5528, .F. ) ;
#7217=CARTESIAN_POINT ( 'NONE',  ( 609.8579287883226243, 189.7296425882048823, 189.8646579186752774 ) ) ;
#7233=DIRECTION ( 'NONE',  ( -1.000000000000000000, 0.000000000000000000, 0.000000000000000000 ) ) ;
#7271=LINE ( 'NONE', #9345, #9715 ) ;
#7277=CARTESIAN_POINT ( 'NONE',  ( 610.7405786874708156, 188.6041887390371130, 185.0905558487023370 ) ) ;
#7286=CARTESIAN_POINT ( 'NONE',  ( 609.6829874266189790, 186.4320250235422805, 187.4339272673398398 ) ) ;
#7306=CIRCLE ( 'NONE', #933, 2.649999999999985700 ) ;
#7308=VERTEX_POINT ( 'NONE', #6843 ) ;
#7328=PLANE ( 'NONE',  #14435 ) ;
#7340=VERTEX_POINT ( 'NONE', #10387 ) ;
#7353=CARTESIAN_POINT ( 'NONE',  ( 142.4540310085880606, 355.9707293956415697, 187.0000000000000000 ) ) ;
#7368=CARTESIAN_POINT ( 'NONE',  ( 610.6294623944595514, 188.6821150189054777, 185.3758453455904771 ) ) ;
#7446=EDGE_CURVE ( 'NONE', #5805, #2398, #2556, .T. ) ;
#7461=PLANE ( 'NONE',  #7076 ) ;
#7494=CARTESIAN_POINT ( 'NONE',  ( 609.7124105659718225, 187.8865375995820557, 188.9268648956065419 ) ) ;
#7507=CARTESIAN_POINT ( 'NONE',  ( 610.0858458365329398, 190.4893660822393144, 186.9132285165672727 ) ) ;
#7538=DIRECTION ( 'NONE',  ( 0.000000000000000000, 0.000000000000000000, 1.000000000000000000 ) ) ;
#7544=APPLICATION_CONTEXT ( 'automotive_design' ) ;
#7548=ORIENTED_EDGE ( 'NONE', *, *, #5185, .F. ) ;
#7551=VERTEX_POINT ( 'NONE', #13612 ) ;
#7579=CARTESIAN_POINT ( 'NONE',  ( 609.8848581100098727, 185.7487647174620520, 185.4822770966949008 ) ) ;
#7590=CARTESIAN_POINT ( 'NONE',  ( 610.8707502976318438, 188.5815814653741427, 184.8000000000000682 ) ) ;
#7620=VERTEX_POINT ( 'NONE', #11326 ) ;
#7624=DIRECTION ( 'NONE',  ( -0.9578262852211513190, 0.2873478855663453846, 0.000000000000000000 ) ) ;
#7654=ORIENTED_EDGE ( 'NONE', *, *, #12631, .F. ) ;
#7656=CARTESIAN_POINT ( 'NONE',  ( 609.7152679600854981, 186.3148376777868975, 187.1062553063055418 ) ) ;
#7690=CARTESIAN_POINT ( 'NONE',  ( -8.074769166705394241, 378.0965165842501392, 187.0000000000000000 ) ) ;
#7704=LINE ( 'NONE', #3139, #13952 ) ;
#7717=CARTESIAN_POINT ( 'NONE',  ( 609.8294541519869654, 189.4056243435263980, 189.7329333695814739 ) ) ;
#7767=ORIENTED_EDGE ( 'NONE', *, *, #704, .F. ) ;
#7803=VECTOR ( 'NONE', #13662, 1000.000000000000227 ) ;
#7808=FACE_OUTER_BOUND ( 'NONE', #5779, .T. ) ;
#7822=LINE ( 'NONE', #12160, #1187 ) ;
#7849=ORIENTED_EDGE ( 'NONE', *, *, #10962, .T. ) ;
#7893=CARTESIAN_POINT ( 'NONE',  ( -8.074769166705396017, 378.0965165842501392, 187.0000000000000284 ) ) ;
#7904=ORIENTED_EDGE ( 'NONE', *, *, #11771, .T. ) ;
#7969=ORIENTED_EDGE ( 'NONE', *, *, #157, .T. ) ;
#7973=CARTESIAN_POINT ( 'NONE',  ( 139.8040310085880833, 355.9707293956415697, 187.0000000000000000 ) ) ;
#8076=VERTEX_POINT ( 'NONE', #12855 ) ;
#8082=ADVANCED_FACE ( 'NONE', ( #2814 ), #4759, .F. ) ;
#8088=PLANE ( 'NONE',  #11296 ) ;
#8130=ORIENTED_EDGE ( 'NONE', *, *, #9009, .F. ) ;
#8160=PRODUCT ( 'sliding track', 'sliding track', '', ( #1171 ) ) ;
#8191=DIRECTION ( 'NONE',  ( 1.003269780210927276E-15, 3.344232600703091053E-15, 1.000000000000000000 ) ) ;
#8206=CARTESIAN_POINT ( 'NONE',  ( 446.3084422793565409, 264.0194060144110608, 190.0000000000000000 ) ) ;
#8244=CARTESIAN_POINT ( 'NONE',  ( 609.9289135522120660, 190.4185930515760958, 190.0000000000000284 ) ) ;
#8302=CARTESIAN_POINT ( 'NONE',  ( -10.00000000000000000, 371.6790804732683569, 190.0000000000000000 ) ) ;
#8329=ORIENTED_EDGE ( 'NONE', *, *, #8917, .F. ) ;
#8351=DIRECTION ( 'NONE',  ( -1.000000000000000000, 0.000000000000000000, 0.000000000000000000 ) ) ;
#8390=CARTESIAN_POINT ( 'NONE',  ( 609.7898554267394502, 185.8834251265051307, 186.1610889986683048 ) ) ;
#8398=ORIENTED_EDGE ( 'NONE', *, *, #12194, .T. ) ;
#8406=UNCERTAINTY_MEASURE_WITH_UNIT (LENGTH_MEASURE( 1.000000000000000082E-05 ), #1077, 'distance_accuracy_value', 'NONE');
#8462=DIRECTION ( 'NONE',  ( -1.000000000000000000, 0.000000000000000000, 0.000000000000000000 ) ) ;
#8467=EDGE_CURVE ( 'NONE', #3014, #2565, #3549, .T. ) ;
#8509=CARTESIAN_POINT ( 'NONE',  ( -8.505790995054899994, 376.6597771564184427, 184.8000000000000398 ) ) ;
#8520=EDGE_LOOP ( 'NONE', ( #7548, #8329, #13332, #13684 ) ) ;
#8522=CARTESIAN_POINT ( 'NONE',  ( -9.999999999999998224, 376.8992337277234128, 187.0000000000000000 ) ) ;
#8561=CARTESIAN_POINT ( 'NONE',  ( -8.505790995054940851, 376.6597771564182722, 190.0000000000000284 ) ) ;
#8586=EDGE_LOOP ( 'NONE', ( #11824, #5309 ) ) ;
#8606=CARTESIAN_POINT ( 'NONE',  ( 609.7206935199311602, 188.0285076711449790, 189.0295014234984023 ) ) ;
#8628=CARTESIAN_POINT ( 'NONE',  ( 0.000000000000000000, 0.000000000000000000, 190.0000000000000000 ) ) ;
#8632=LINE ( 'NONE', #12022, #8647 ) ;
#8647=VECTOR ( 'NONE', #12098, 1000.000000000000114 ) ;
#8655=CARTESIAN_POINT ( 'NONE',  ( -9.999999999999957367, 376.8992337277236970, 187.0000000000000000 ) ) ;
#8688=AXIS2_PLACEMENT_3D ( 'NONE', #4444, #9773, #10422 ) ;
#8752=VERTEX_POINT ( 'NONE', #6826 ) ;
#8773=CARTESIAN_POINT ( 'NONE',  ( 610.6379424248335681, 188.7103817868187150, 185.3679143846944157 ) ) ;
#8784=VECTOR ( 'NONE', #13641, 1000.000000000000114 ) ;
#8821=EDGE_LOOP ( 'NONE', ( #1168, #4845, #9291, #5840 ) ) ;
#8874=ORIENTED_EDGE ( 'NONE', *, *, #7446, .F. ) ;
#8887=CARTESIAN_POINT ( 'NONE',  ( 609.7735223591643035, 188.7684563956151464, 189.4730470240896807 ) ) ;
#8902=ADVANCED_FACE ( 'NONE', ( #14131 ), #1514, .F. ) ;
#8903=AXIS2_PLACEMENT_3D ( 'NONE', #4774, #6005, #4988 ) ;
#8905=PLANE ( 'NONE',  #6437 ) ;
#8907=ORIENTED_EDGE ( 'NONE', *, *, #8467, .F. ) ;
#8909=EDGE_CURVE ( 'NONE', #6858, #12823, #9630, .T. ) ;
#8914=VECTOR ( 'NONE', #3788, 1000.000000000000000 ) ;
#8917=EDGE_CURVE ( 'NONE', #2870, #12209, #1575, .T. ) ;
#8958=VECTOR ( 'NONE', #13042, 1000.000000000000114 ) ;
#8968=ORIENTED_EDGE ( 'NONE', *, *, #12194, .F. ) ;
#8988=EDGE_CURVE ( 'NONE', #3959, #2398, #11903, .T. ) ;
#9009=EDGE_CURVE ( 'NONE', #11318, #2694, #7704, .T. ) ;
#9012=ORIENTED_EDGE ( 'NONE', *, *, #4856, .T. ) ;
#9042=ORIENTED_EDGE ( 'NONE', *, *, #11509, .F. ) ;
#9059=SURFACE_STYLE_USAGE ( .BOTH. , #12369 ) ;
#9063=ORIENTED_EDGE ( 'NONE', *, *, #9009, .T. ) ;
#9128=ORIENTED_EDGE ( 'NONE', *, *, #10451, .T. ) ;
#9143=CARTESIAN_POINT ( 'NONE',  ( 610.2669374424701800, 189.5106555248625284, 186.4579326193729969 ) ) ;
#9159=ORIENTED_EDGE ( 'NONE', *, *, #8988, .F. ) ;
#9166=ORIENTED_EDGE ( 'NONE', *, *, #11771, .F. ) ;
#9193=EDGE_CURVE ( 'NONE', #9351, #2694, #14182, .T. ) ;
#9204=( NAMED_UNIT ( * ) PLANE_ANGLE_UNIT ( ) SI_UNIT ( $, .RADIAN. ) );
#9227=FACE_OUTER_BOUND ( 'NONE', #10545, .T. ) ;
#9229=ORIENTED_EDGE ( 'NONE', *, *, #3222, .F. ) ;
#9254=EDGE_CURVE ( 'NONE', #6357, #8076, #3106, .T. ) ;
#9288=CARTESIAN_POINT ( 'NONE',  ( 448.9584422793565750, 264.0194060144110608, 190.0000000000000000 ) ) ;
#9291=ORIENTED_EDGE ( 'NONE', *, *, #3222, .T. ) ;
#9292=DIRECTION ( 'NONE',  ( -0.000000000000000000, -0.000000000000000000, -1.000000000000000000 ) ) ;
#9310=AXIS2_PLACEMENT_3D ( 'NONE', #5986, #2731, #7233 ) ;
#9327=FACE_OUTER_BOUND ( 'NONE', #13594, .T. ) ;
#9345=CARTESIAN_POINT ( 'NONE',  ( -10.00000000000000888, 371.6790804732683569, 169.9999999999999716 ) ) ;
#9351=VERTEX_POINT ( 'NONE', #6065 ) ;
#9361=CARTESIAN_POINT ( 'NONE',  ( 609.9913795634330427, 185.6503456847118514, 184.8000000000000966 ) ) ;
#9371=ORIENTED_EDGE ( 'NONE', *, *, #847, .T. ) ;
#9372=( NAMED_UNIT ( * ) SI_UNIT ( $, .STERADIAN. ) SOLID_ANGLE_UNIT ( ) );
#9395=CIRCLE ( 'NONE', #3029, 2.649999999999985700 ) ;
#9420=CARTESIAN_POINT ( 'NONE',  ( -9.999999999999998224, 376.8992337277234128, 187.0000000000000000 ) ) ;
#9429=AXIS2_PLACEMENT_3D ( 'NONE', #7184, #11674, #1503 ) ;
#9437=CARTESIAN_POINT ( 'NONE',  ( 609.6767525226840689, 186.8636552924789669, 187.9956429438695977 ) ) ;
#9440=AXIS2_PLACEMENT_3D ( 'NONE', #4347, #14302, #6417 ) ;
#9445=EDGE_CURVE ( 'NONE', #12510, #7620, #3081, .T. ) ;
#9474=VECTOR ( 'NONE', #1898, 1000.000000000000114 ) ;
#9480=PLANE ( 'NONE',  #688 ) ;
#9484=CARTESIAN_POINT ( 'NONE',  ( 103.3965373855728558, 344.6551246185656510, 190.0000000000000000 ) ) ;
#9518=FACE_OUTER_BOUND ( 'NONE', #8821, .T. ) ;
#9532=LINE ( 'NONE', #4202, #4006 ) ;
#9578=ADVANCED_FACE ( 'NONE', ( #10998 ), #7461, .T. ) ;
#9583=CARTESIAN_POINT ( 'NONE',  ( 610.3661002516460030, 189.1614810556852717, 186.1520027839448232 ) ) ;
#9595=EDGE_CURVE ( 'NONE', #7620, #12510, #7306, .T. ) ;
#9630=LINE ( 'NONE', #8522, #12513 ) ;
#9632=EDGE_CURVE ( 'NONE', #2694, #5396, #11437, .T. ) ;
#9637=ORIENTED_EDGE ( 'NONE', *, *, #8467, .T. ) ;
#9640=VECTOR ( 'NONE', #12790, 1000.000000000000000 ) ;
#9659=CARTESIAN_POINT ( 'NONE',  ( 610.7375075899259400, 188.5899201489639267, 185.0880224589102454 ) ) ;
#9670=ORIENTED_EDGE ( 'NONE', *, *, #4729, .F. ) ;
#9694=AXIS2_PLACEMENT_3D ( 'NONE', #7973, #2366, #6874 ) ;
#9706=LINE ( 'NONE', #1791, #11040 ) ;
#9715=VECTOR ( 'NONE', #1666, 1000.000000000000114 ) ;
#9773=DIRECTION ( 'NONE',  ( -0.000000000000000000, -0.000000000000000000, -1.000000000000000000 ) ) ;
#9778=EDGE_LOOP ( 'NONE', ( #1463, #8398, #5127, #13803 ) ) ;
#9782=ORIENTED_EDGE ( 'NONE', *, *, #3414, .F. ) ;
#9812=DIRECTION ( 'NONE',  ( -0.000000000000000000, 0.000000000000000000, -1.000000000000000000 ) ) ;
#9839=CARTESIAN_POINT ( 'NONE',  ( 610.0000000000000000, 227.4403065089105951, 187.0000000000000000 ) ) ;
#9856=CARTESIAN_POINT ( 'NONE',  ( 610.0000000000000000, 227.4403065089105951, 187.0000000000000000 ) ) ;
#9939=CARTESIAN_POINT ( 'NONE',  ( 609.6990795428844194, 187.6157354204721912, 188.7107384553189888 ) ) ;
#9973=AXIS2_PLACEMENT_3D ( 'NONE', #8509, #13234, #967 ) ;
#9994=EDGE_CURVE ( 'NONE', #12104, #8752, #5910, .T. ) ;
#10049=ORIENTED_EDGE ( 'NONE', *, *, #9193, .T. ) ;
#10060=ORIENTED_EDGE ( 'NONE', *, *, #3848, .T. ) ;
#10081=DIRECTION ( 'NONE',  ( -1.000000000000000000, 0.000000000000000000, 0.000000000000000000 ) ) ;
#10084=EDGE_CURVE ( 'NONE', #8076, #6357, #12500, .T. ) ;
#10163=FACE_BOUND ( 'NONE', #5438, .T. ) ;
#10166=FILL_AREA_STYLE ('',( #2415 ) ) ;
#10174=PLANE ( 'NONE',  #4925 ) ;
#10211=DIRECTION ( 'NONE',  ( -1.000000000000000000, 0.000000000000000000, 0.000000000000000000 ) ) ;
#10234=CARTESIAN_POINT ( 'NONE',  ( 0.000000000000000000, 0.000000000000000000, 187.0000000000000000 ) ) ;
#10282=ORIENTED_EDGE ( 'NONE', *, *, #4729, .T. ) ;
#10302=PRESENTATION_STYLE_ASSIGNMENT (( #9059 ) ) ;
#10304=ORIENTED_EDGE ( 'NONE', *, *, #1011, .T. ) ;
#10310=ORIENTED_EDGE ( 'NONE', *, *, #2953, .T. ) ;
#10384=VECTOR ( 'NONE', #10955, 1000.000000000000000 ) ;
#10387=CARTESIAN_POINT ( 'NONE',  ( -10.00000000000000000, 413.4403065089105667, 187.0000000000000000 ) ) ;
#10392=DIRECTION ( 'NONE',  ( 0.9578262852211489875, -0.2873478855663534892, 0.000000000000000000 ) ) ;
#10422=DIRECTION ( 'NONE',  ( -1.000000000000000000, 0.000000000000000000, 0.000000000000000000 ) ) ;
#10429=CARTESIAN_POINT ( 'NONE',  ( 139.8040310085880833, 355.9707293956415697, 190.0000000000000000 ) ) ;
#10435=CIRCLE ( 'NONE', #9973, 2.199999999999984635 ) ;
#10451=EDGE_CURVE ( 'NONE', #7620, #8076, #11277, .T. ) ;
#10471=CARTESIAN_POINT ( 'NONE',  ( 609.8556724072889210, 189.7221213180926611, 189.8938770989753095 ) ) ;
#10510=DIRECTION ( 'NONE',  ( -0.000000000000000000, -0.000000000000000000, -1.000000000000000000 ) ) ;
#10545=EDGE_LOOP ( 'NONE', ( #8968, #6734, #9128, #12324 ) ) ;
#10560=CARTESIAN_POINT ( 'NONE',  ( 610.0000000000001137, 185.6790804732683853, 169.9999999999999716 ) ) ;
#10592=FACE_OUTER_BOUND ( 'NONE', #4938, .T. ) ;
#10644=ADVANCED_FACE ( 'NONE', ( #9518 ), #4524, .F. ) ;
#10654=ORIENTED_EDGE ( 'NONE', *, *, #11531, .T. ) ;
#10691=CARTESIAN_POINT ( 'NONE',  ( 610.1796992002056186, 189.8973840637093247, 186.7223300543793698 ) ) ;
#10706=EDGE_CURVE ( 'NONE', #11318, #11200, #13191, .T. ) ;
#10751=LINE ( 'NONE', #627, #6639 ) ;
#10782=LINE ( 'NONE', #2817, #12671 ) ;
#10822=DIRECTION ( 'NONE',  ( -1.000000000000000000, 0.000000000000000000, 0.000000000000000000 ) ) ;
#10824=ORIENTED_EDGE ( 'NONE', *, *, #9193, .F. ) ;
#10904=ORIENTED_EDGE ( 'NONE', *, *, #12485, .T. ) ;
#10913=CARTESIAN_POINT ( 'NONE',  ( 610.3730626637085379, 189.1846890958936740, 186.1333820183295984 ) ) ;
#10937=DIRECTION ( 'NONE',  ( 0.2873478855663452736, 0.9578262852211513190, -3.491481338843133355E-15 ) ) ;
#10955=DIRECTION ( 'NONE',  ( 0.000000000000000000, -1.000000000000000000, 0.000000000000000000 ) ) ;
#10962=EDGE_CURVE ( 'NONE', #13246, #12104, #7271, .T. ) ;
#10964=LINE ( 'NONE', #9856, #5403 ) ;
#10977=CARTESIAN_POINT ( 'NONE',  ( 443.6584422793565636, 264.0194060144110608, 187.0000000000000000 ) ) ;
#10997=CARTESIAN_POINT ( 'NONE',  ( 448.9584422793565750, 264.0194060144110608, 187.0000000000000000 ) ) ;
#10998=FACE_OUTER_BOUND ( 'NONE', #8520, .T. ) ;
#11040=VECTOR ( 'NONE', #5412, 1000.000000000000000 ) ;
#11045=DIRECTION ( 'NONE',  ( 0.9578262852211514300, -0.2873478855663453846, -1.407442229263725984E-15 ) ) ;
#11072=EDGE_LOOP ( 'NONE', ( #10654, #9159, #1121, #13308 ) ) ;
#11082=UNCERTAINTY_MEASURE_WITH_UNIT (LENGTH_MEASURE( 1.000000000000000082E-05 ), #12770, 'distance_accuracy_value', 'NONE');
#11109=CARTESIAN_POINT ( 'NONE',  ( -9.137956343301000928, 374.5525593289319204, 169.9999999999999716 ) ) ;
#11114=CARTESIAN_POINT ( 'NONE',  ( 609.7493509738548028, 188.4639666770506494, 189.3135794259398494 ) ) ;
#11125=CARTESIAN_POINT ( 'NONE',  ( 610.8620436566991430, 188.5525593289319488, 184.8000000000000682 ) ) ;
#11154=DIRECTION ( 'NONE',  ( -0.9578262852211513190, 0.2873478855663453846, 0.000000000000000000 ) ) ;
#11159=CLOSED_SHELL ( 'NONE', ( #8902, #572, #11438, #13771, #13680, #3919, #12429, #2262, #2959, #13312, #10644, #14166, #6703, #102, #11859, #8082, #3672, #9578, #12821, #13131, #1560 ) ) ;
#11163=LINE ( 'NONE', #5550, #13634 ) ;
#11191=EDGE_LOOP ( 'NONE', ( #5609, #2166 ) ) ;
#11193=DIRECTION ( 'NONE',  ( -0.000000000000000000, 0.000000000000000000, -1.000000000000000000 ) ) ;
#11200=VERTEX_POINT ( 'NONE', #5781 ) ;
#11277=LINE ( 'NONE', #2263, #729 ) ;
#11279=CARTESIAN_POINT ( 'NONE',  ( 610.0000000000001137, 185.6790804732684421, 184.8000000000000682 ) ) ;
#11296=AXIS2_PLACEMENT_3D ( 'NONE', #10234, #11193, #10081 ) ;
#11318=VERTEX_POINT ( 'NONE', #6075 ) ;
#11326=CARTESIAN_POINT ( 'NONE',  ( 137.1540310085880776, 355.9707293956415697, 190.0000000000000000 ) ) ;
#11345=ORIENTED_EDGE ( 'NONE', *, *, #12601, .F. ) ;
#11370=ORIENTED_EDGE ( 'NONE', *, *, #966, .F. ) ;
#11371=EDGE_LOOP ( 'NONE', ( #11647, #1909, #374, #7849 ) ) ;
#11381=DIRECTION ( 'NONE',  ( -1.000000000000000000, 0.000000000000000000, 0.000000000000000000 ) ) ;
#11436=( NAMED_UNIT ( * ) PLANE_ANGLE_UNIT ( ) SI_UNIT ( $, .RADIAN. ) );
#11437=LINE ( 'NONE', #2140, #3312 ) ;
#11438=ADVANCED_FACE ( 'NONE', ( #5118 ), #7328, .F. ) ;
#11460=FACE_OUTER_BOUND ( 'NONE', #2001, .T. ) ;
#11463=ORIENTED_EDGE ( 'NONE', *, *, #8917, .T. ) ;
#11486=VECTOR ( 'NONE', #10937, 1000.000000000000114 ) ;
#11497=CARTESIAN_POINT ( 'NONE',  ( 610.0421465541240877, 190.7920056415575516, 186.9999999999999432 ) ) ;
#11509=EDGE_CURVE ( 'NONE', #3640, #11318, #11571, .T. ) ;
#11519=CARTESIAN_POINT ( 'NONE',  ( 610.0000000000001137, 185.6790804732684421, 187.0000000000000000 ) ) ;
#11531=EDGE_CURVE ( 'NONE', #2870, #2398, #12380, .T. ) ;
#11571=LINE ( 'NONE', #7893, #8784 ) ;
#11576=AXIS2_PLACEMENT_3D ( 'NONE', #13534, #12482, #5776 ) ;
#11604=LINE ( 'NONE', #5997, #9640 ) ;
#11647=ORIENTED_EDGE ( 'NONE', *, *, #9994, .T. ) ;
#11672=DIRECTION ( 'NONE',  ( -1.000000000000000000, 0.000000000000000000, 0.000000000000000000 ) ) ;
#11674=DIRECTION ( 'NONE',  ( 0.9578262852211514300, -0.2873478855663454401, -0.000000000000000000 ) ) ;
#11691=LINE ( 'NONE', #9420, #13440 ) ;
#11703=CARTESIAN_POINT ( 'NONE',  ( 610.0000000000001137, 191.1080398579019288, 190.0300000000000296 ) ) ;
#11757=AXIS2_PLACEMENT_3D ( 'NONE', #8628, #9812, #511 ) ;
#11771=EDGE_CURVE ( 'NONE', #2441, #13081, #6488, .T. ) ;
#11824=ORIENTED_EDGE ( 'NONE', *, *, #77, .T. ) ;
#11853=CARTESIAN_POINT ( 'NONE',  ( 610.3331342679523459, 189.2775297294220991, 186.2537089296249349 ) ) ;
#11859=ADVANCED_FACE ( 'NONE', ( #12213 ), #8905, .F. ) ;
#11903=LINE ( 'NONE', #4996, #5697 ) ;
#11905=LINE ( 'NONE', #8302, #13919 ) ;
#11951=DIRECTION ( 'NONE',  ( 0.2873478855663454401, 0.9578262852211514300, -3.831370512995697396E-15 ) ) ;
#11986=AXIS2_PLACEMENT_3D ( 'NONE', #10560, #8191, #12702 ) ;
#11991=CARTESIAN_POINT ( 'NONE',  ( 609.9372209285376130, 185.6979141947072378, 185.1431837845556743 ) ) ;
#12022=CARTESIAN_POINT ( 'NONE',  ( -9.511508594537124495, 378.5275384125996538, 187.0000000000000284 ) ) ;
#12033=CARTESIAN_POINT ( 'NONE',  ( 102.3333502089745650, 341.1111673632485122, -1.352973838917536986E-12 ) ) ;
#12086=ORIENTED_EDGE ( 'NONE', *, *, #966, .T. ) ;
#12098=DIRECTION ( 'NONE',  ( 0.9578262852211489875, -0.2873478855663534892, 0.000000000000000000 ) ) ;
#12104=VERTEX_POINT ( 'NONE', #11109 ) ;
#12107=DIRECTION ( 'NONE',  ( -1.000000000000000000, 0.000000000000000000, 0.000000000000000000 ) ) ;
#12133=LINE ( 'NONE', #14169, #2783 ) ;
#12149=CARTESIAN_POINT ( 'NONE',  ( -8.505790995055066972, 376.6597771564184427, 187.0000000000000284 ) ) ;
#12152=CARTESIAN_POINT ( 'NONE',  ( -10.00000000000003730, 371.6790804732684137, 169.9999999999999716 ) ) ;
#12158=CARTESIAN_POINT ( 'NONE',  ( 610.0000000000002274, 185.6790804732683284, 169.9999999999999716 ) ) ;
#12160=CARTESIAN_POINT ( 'NONE',  ( 610.8620436566991430, 188.5525593289318920, 187.0000000000000000 ) ) ;
#12185=ORIENTED_EDGE ( 'NONE', *, *, #10706, .T. ) ;
#12194=EDGE_CURVE ( 'NONE', #12510, #6357, #3284, .T. ) ;
#12209=VERTEX_POINT ( 'NONE', #12498 ) ;
#12213=FACE_OUTER_BOUND ( 'NONE', #2708, .T. ) ;
#12250=PLANE ( 'NONE',  #6592 ) ;
#12286=ORIENTED_EDGE ( 'NONE', *, *, #13907, .T. ) ;
#12313=DIRECTION ( 'NONE',  ( -1.000000000000000000, 0.000000000000000000, -0.000000000000000000 ) ) ;
#12322=AXIS2_PLACEMENT_3D ( 'NONE', #8206, #3877, #11672 ) ;
#12324=ORIENTED_EDGE ( 'NONE', *, *, #10084, .T. ) ;
#12369=SURFACE_SIDE_STYLE ('',( #2327 ) ) ;
#12370=ORIENTED_EDGE ( 'NONE', *, *, #12485, .F. ) ;
#12380=LINE ( 'NONE', #11279, #983 ) ;
#12399=LINE ( 'NONE', #6879, #3744 ) ;
#12429=ADVANCED_FACE ( 'NONE', ( #13304 ), #13239, .F. ) ;
#12482=DIRECTION ( 'NONE',  ( -0.9578262852211514300, 0.2873478855663454401, 0.000000000000000000 ) ) ;
#12485=EDGE_CURVE ( 'NONE', #6858, #7340, #9706, .T. ) ;
#12498=CARTESIAN_POINT ( 'NONE',  ( -9.137956343300853490, 374.5525593289319204, 184.8000000000000398 ) ) ;
#12500=CIRCLE ( 'NONE', #9694, 2.649999999999985700 ) ;
#12509=STYLED_ITEM ( 'NONE', ( #10302 ), #6538 ) ;
#12510=VERTEX_POINT ( 'NONE', #6376 ) ;
#12513=VECTOR ( 'NONE', #1733, 1000.000000000000000 ) ;
#12529=ORIENTED_EDGE ( 'NONE', *, *, #6463, .F. ) ;
#12550=VECTOR ( 'NONE', #5370, 1000.000000000000000 ) ;
#12555=EDGE_CURVE ( 'NONE', #3640, #5396, #11163, .T. ) ;
#12601=EDGE_CURVE ( 'NONE', #13081, #2565, #3984, .T. ) ;
#12614=CARTESIAN_POINT ( 'NONE',  ( 610.2366331756301179, 189.6374102278066971, 186.5502271136477361 ) ) ;
#12631=EDGE_CURVE ( 'NONE', #3596, #11200, #12399, .T. ) ;
#12667=DIRECTION ( 'NONE',  ( -1.000000000000000000, 0.000000000000000000, 0.000000000000000000 ) ) ;
#12671=VECTOR ( 'NONE', #7538, 1000.000000000000000 ) ;
#12699=EDGE_CURVE ( 'NONE', #7340, #5137, #13973, .T. ) ;
#12702=DIRECTION ( 'NONE',  ( 0.000000000000000000, -1.000000000000000000, 3.344232600703091053E-15 ) ) ;
#12724=ORIENTED_EDGE ( 'NONE', *, *, #12699, .F. ) ;
#12756=ORIENTED_EDGE ( 'NONE', *, *, #2429, .F. ) ;
#12757=CARTESIAN_POINT ( 'NONE',  ( 609.7455576527837593, 188.4502455723027481, 189.3436892194421546 ) ) ;
#12765=EDGE_LOOP ( 'NONE', ( #4121, #2537, #12756, #6988 ) ) ;
#12770=( LENGTH_UNIT ( ) NAMED_UNIT ( * ) SI_UNIT ( .MILLI., .METRE. ) );
#12790=DIRECTION ( 'NONE',  ( -0.000000000000000000, -0.000000000000000000, 1.000000000000000000 ) ) ;
#12798=DIRECTION ( 'NONE',  ( -0.9578262852211489875, 0.2873478855663534892, 0.000000000000000000 ) ) ;
#12821=ADVANCED_FACE ( 'NONE', ( #4890 ), #3709, .F. ) ;
#12823=VERTEX_POINT ( 'NONE', #4968 ) ;
#12850=FACE_OUTER_BOUND ( 'NONE', #9778, .T. ) ;
#12855=CARTESIAN_POINT ( 'NONE',  ( 137.1540310085880776, 355.9707293956415697, 187.0000000000000000 ) ) ;
#12904=LINE ( 'NONE', #268, #1220 ) ;
#12909=EDGE_LOOP ( 'NONE', ( #1600, #2480 ) ) ;
#12993=MECHANICAL_DESIGN_GEOMETRIC_PRESENTATION_REPRESENTATION('',(#12509),#5226);
#13042=DIRECTION ( 'NONE',  ( 0.9578262852211513190, -0.2873478855663453291, -0.000000000000000000 ) ) ;
#13049=CARTESIAN_POINT ( 'NONE',  ( 610.0000000000001137, 191.1080398579018720, 187.0000000000000000 ) ) ;
#13057=CARTESIAN_POINT ( 'NONE',  ( 610.0429133068968213, 190.7986032820865319, 186.9697000000000173 ) ) ;
#13081=VERTEX_POINT ( 'NONE', #1808 ) ;
#13107=LINE ( 'NONE', #6534, #644 ) ;
#13131=ADVANCED_FACE ( 'NONE', ( #9227 ), #14013, .F. ) ;
#13136=EDGE_CURVE ( 'NONE', #11200, #2870, #6066, .T. ) ;
#13172=ORIENTED_EDGE ( 'NONE', *, *, #9632, .T. ) ;
#13191=LINE ( 'NONE', #12149, #9474 ) ;
#13212=AXIS2_PLACEMENT_3D ( 'NONE', #10429, #3870, #8351 ) ;
#13223=ORIENTED_EDGE ( 'NONE', *, *, #1011, .F. ) ;
#13234=DIRECTION ( 'NONE',  ( -0.9578262852211514300, 0.2873478855663454401, 0.000000000000000000 ) ) ;
#13235=EDGE_CURVE ( 'NONE', #7340, #3596, #10964, .T. ) ;
#13239=PLANE ( 'NONE',  #2796 ) ;
#13246=VERTEX_POINT ( 'NONE', #5296 ) ;
#13256=CARTESIAN_POINT ( 'NONE',  ( 610.0000000000000000, 227.4403065089105951, 190.0000000000000000 ) ) ;
#13270=ORIENTED_EDGE ( 'NONE', *, *, #12601, .T. ) ;
#13304=FACE_OUTER_BOUND ( 'NONE', #5964, .T. ) ;
#13308=ORIENTED_EDGE ( 'NONE', *, *, #5215, .T. ) ;
#13312=ADVANCED_FACE ( 'NONE', ( #2684 ), #9480, .T. ) ;
#13325=CARTESIAN_POINT ( 'NONE',  ( 609.9288325809317257, 190.4177448864037956, 189.9663414180174925 ) ) ;
#13332=ORIENTED_EDGE ( 'NONE', *, *, #5215, .F. ) ;
#13377=APPLICATION_CONTEXT ( 'automotive_design' ) ;
#13410=VERTEX_POINT ( 'NONE', #6549 ) ;
#13435=ORIENTED_EDGE ( 'NONE', *, *, #58, .F. ) ;
#13440=VECTOR ( 'NONE', #1585, 1000.000000000000000 ) ;
#13442=PRODUCT_DEFINITION ( 'UNKNOWN', '', #3845, #3107 ) ;
#13534=CARTESIAN_POINT ( 'NONE',  ( -8.505790995054894665, 376.6597771564184427, 184.8000000000000398 ) ) ;
#13535=LINE ( 'NONE', #981, #14586 ) ;
#13594=EDGE_LOOP ( 'NONE', ( #12185, #4167, #11463, #7969 ) ) ;
#13601=EDGE_LOOP ( 'NONE', ( #6167, #13435, #4954, #10304, #3519, #2156, #9670 ) ) ;
#13612=CARTESIAN_POINT ( 'NONE',  ( 610.0000000000000000, 227.4403065089105951, 190.0000000000000000 ) ) ;
#13634=VECTOR ( 'NONE', #64, 1000.000000000000000 ) ;
#13641=DIRECTION ( 'NONE',  ( -0.2873478855663437193, -0.9578262852211517631, 0.000000000000000000 ) ) ;
#13649=CARTESIAN_POINT ( 'NONE',  ( 610.7992194312785159, 188.5714065965581483, 184.9452975700425554 ) ) ;
#13662=DIRECTION ( 'NONE',  ( 0.9578262852211513190, -0.2873478855663454401, 2.126837879698859960E-31 ) ) ;
#13667=DIRECTION ( 'NONE',  ( -0.000000000000000000, -0.000000000000000000, -1.000000000000000000 ) ) ;
#13680=ADVANCED_FACE ( 'NONE', ( #10163, #6699, #7808 ), #8088, .T. ) ;
#13684=ORIENTED_EDGE ( 'NONE', *, *, #9994, .F. ) ;
#13709=CIRCLE ( 'NONE', #13943, 2.649999999999985700 ) ;
#13719=DIRECTION ( 'NONE',  ( -0.000000000000000000, -0.000000000000000000, -1.000000000000000000 ) ) ;
#13745=VECTOR ( 'NONE', #5854, 1000.000000000000000 ) ;
#13764=CYLINDRICAL_SURFACE ( 'NONE', #8903, 5.199999999999999289 ) ;
#13771=ADVANCED_FACE ( 'NONE', ( #2475 ), #5007, .F. ) ;
#13781=EDGE_CURVE ( 'NONE', #6858, #7308, #11691, .T. ) ;
#13803=ORIENTED_EDGE ( 'NONE', *, *, #10451, .F. ) ;
#13823=DIRECTION ( 'NONE',  ( -0.2873478855663452736, -0.9578262852211514300, 0.000000000000000000 ) ) ;
#13865=DIRECTION ( 'NONE',  ( 0.9578262852211513190, -0.2873478855663453846, 8.575812866481462478E-17 ) ) ;
#13870=STYLED_ITEM('',(#14667),#2617);
#13907=EDGE_CURVE ( 'NONE', #5137, #7551, #3070, .T. ) ;
#13919=VECTOR ( 'NONE', #7128, 1000.000000000000000 ) ;
#13926=CARTESIAN_POINT ( 'NONE',  ( -9.999999999999998224, 376.8992337277234128, 187.0000000000000000 ) ) ;
#13943=AXIS2_PLACEMENT_3D ( 'NONE', #6325, #14079, #8462 ) ;
#13946=CARTESIAN_POINT ( 'NONE',  ( 610.0000000000001137, 185.6790804732684990, 184.8000000000000966 ) ) ;
#13952=VECTOR ( 'NONE', #2076, 1000.000000000000000 ) ;
#13955=ORIENTED_EDGE ( 'NONE', *, *, #10962, .F. ) ;
#13973=LINE ( 'NONE', #5046, #8914 ) ;
#13998=ORIENTED_EDGE ( 'NONE', *, *, #13235, .F. ) ;
#14013=CYLINDRICAL_SURFACE ( 'NONE', #1142, 2.649999999999985700 ) ;
#14019=CARTESIAN_POINT ( 'NONE',  ( 609.7814593570623174, 185.8554382275811463, 186.1689414351991161 ) ) ;
#14067=DIRECTION ( 'NONE',  ( 0.2873478855663470499, 0.9578262852211508749, 0.000000000000000000 ) ) ;
#14079=DIRECTION ( 'NONE',  ( -0.000000000000000000, -0.000000000000000000, -1.000000000000000000 ) ) ;
#14131=FACE_OUTER_BOUND ( 'NONE', #2009, .T. ) ;
#14138=PLANE ( 'NONE',  #4419 ) ;
#14152=CARTESIAN_POINT ( 'NONE',  ( 610.6325945170714249, 188.6953700521320911, 185.3721572044278787 ) ) ;
#14166=ADVANCED_FACE ( 'NONE', ( #6002 ), #4836, .F. ) ;
#14169=CARTESIAN_POINT ( 'NONE',  ( -8.505790995055079406, 376.6597771564183859, 190.0000000000000284 ) ) ;
#14182=CIRCLE ( 'NONE', #11576, 5.199999999999999289 ) ;
#14240=DIRECTION ( 'NONE',  ( 0.2873478855663453291, 0.9578262852211513190, 0.000000000000000000 ) ) ;
#14290=CARTESIAN_POINT ( 'NONE',  ( 610.0000000000001137, 185.6790804732684705, 184.8000000000000398 ) ) ;
#14299=CARTESIAN_POINT ( 'NONE',  ( 610.0000000000001137, 191.1080398579019572, 186.9697000000000173 ) ) ;
#14302=DIRECTION ( 'NONE',  ( 0.000000000000000000, 0.000000000000000000, 1.000000000000000000 ) ) ;
#14329=CARTESIAN_POINT ( 'NONE',  ( 443.6584422793565636, 264.0194060144110608, 190.0000000000000000 ) ) ;
#14373=CARTESIAN_POINT ( 'NONE',  ( 610.2394425817745969, 189.6441153868865399, 186.5350371479513569 ) ) ;
#14409=AXIS2_PLACEMENT_3D ( 'NONE', #3734, #10510, #378 ) ;
#14430=SHAPE_REPRESENTATION ( 'sliding track', ( #9440 ), #1445 ) ;
#14435=AXIS2_PLACEMENT_3D ( 'NONE', #943, #12313, #1087 ) ;
#14454=ORIENTED_EDGE ( 'NONE', *, *, #8988, .T. ) ;
#14553=CYLINDRICAL_SURFACE ( 'NONE', #8688, 2.649999999999985700 ) ;
#14567=ORIENTED_EDGE ( 'NONE', *, *, #6463, .T. ) ;
#14586=VECTOR ( 'NONE', #2383, 1000.000000000000000 ) ;
#14661=COLOUR_RGB('Sky Blue',0.24,0.69,0.87);
#14662=FILL_AREA_STYLE_COLOUR('',#14661);
#14663=FILL_AREA_STYLE('',(#14662));
#14664=SURFACE_STYLE_FILL_AREA(#14663);
#14665=SURFACE_SIDE_STYLE('',(#14664));
#14666=SURFACE_STYLE_USAGE(.BOTH.,#14665);
#14667=PRESENTATION_STYLE_ASSIGNMENT((#14666));
ENDSEC;
END-ISO-10303-21;
